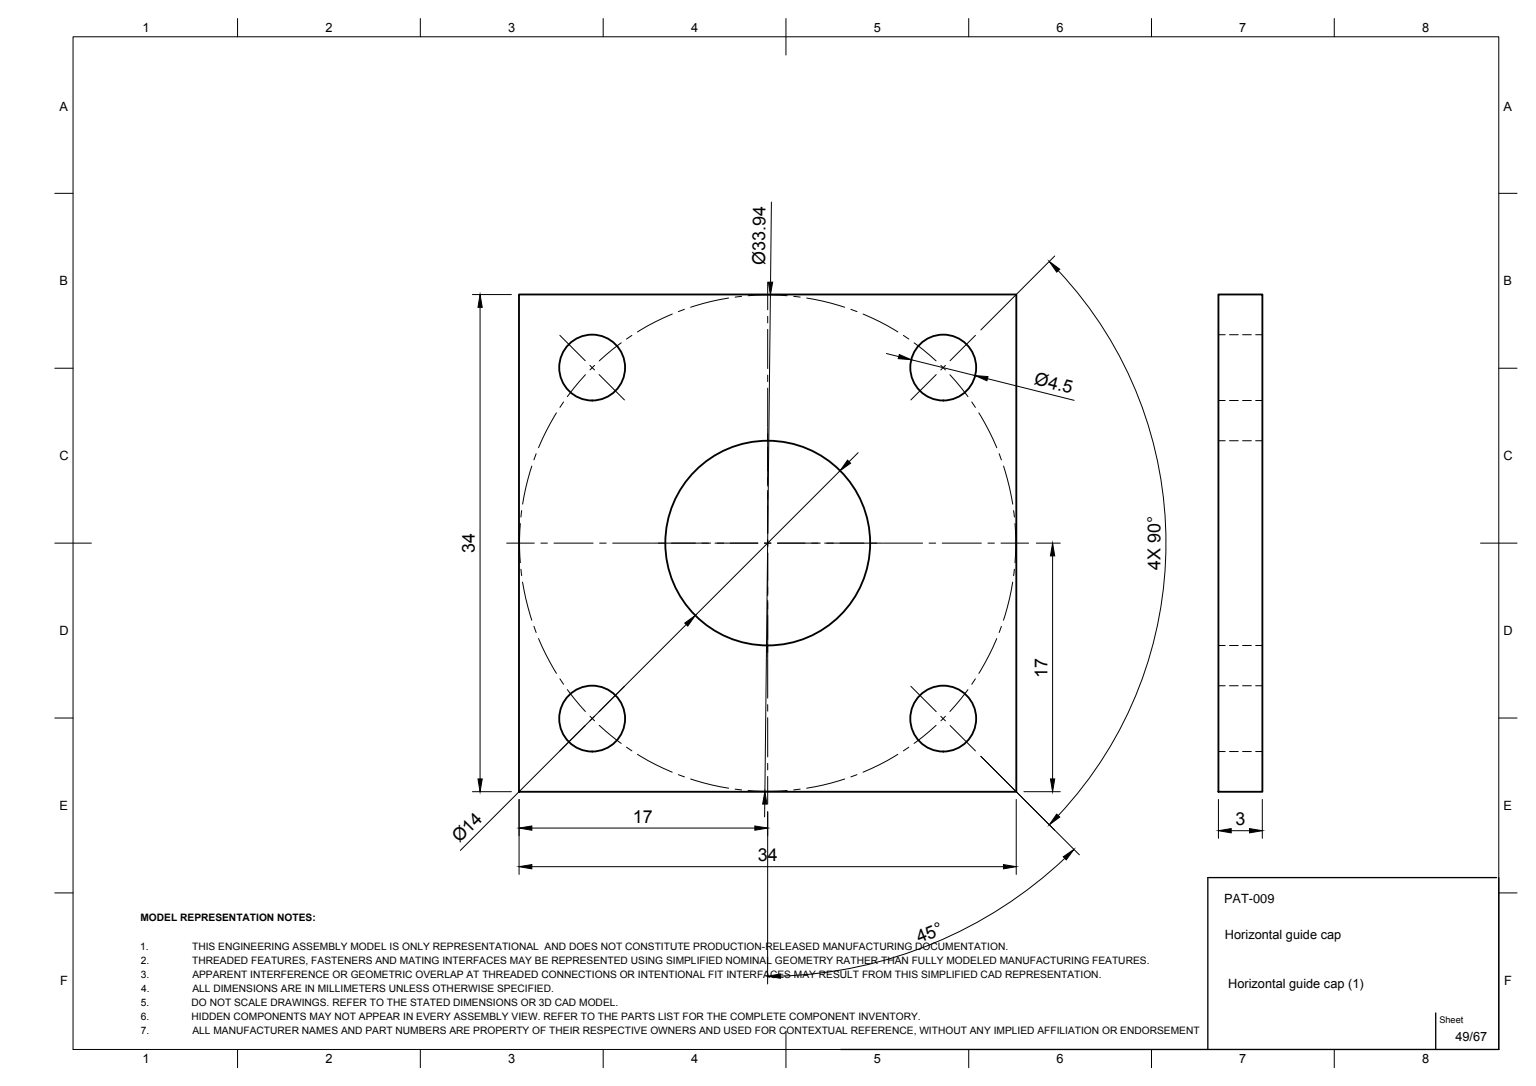
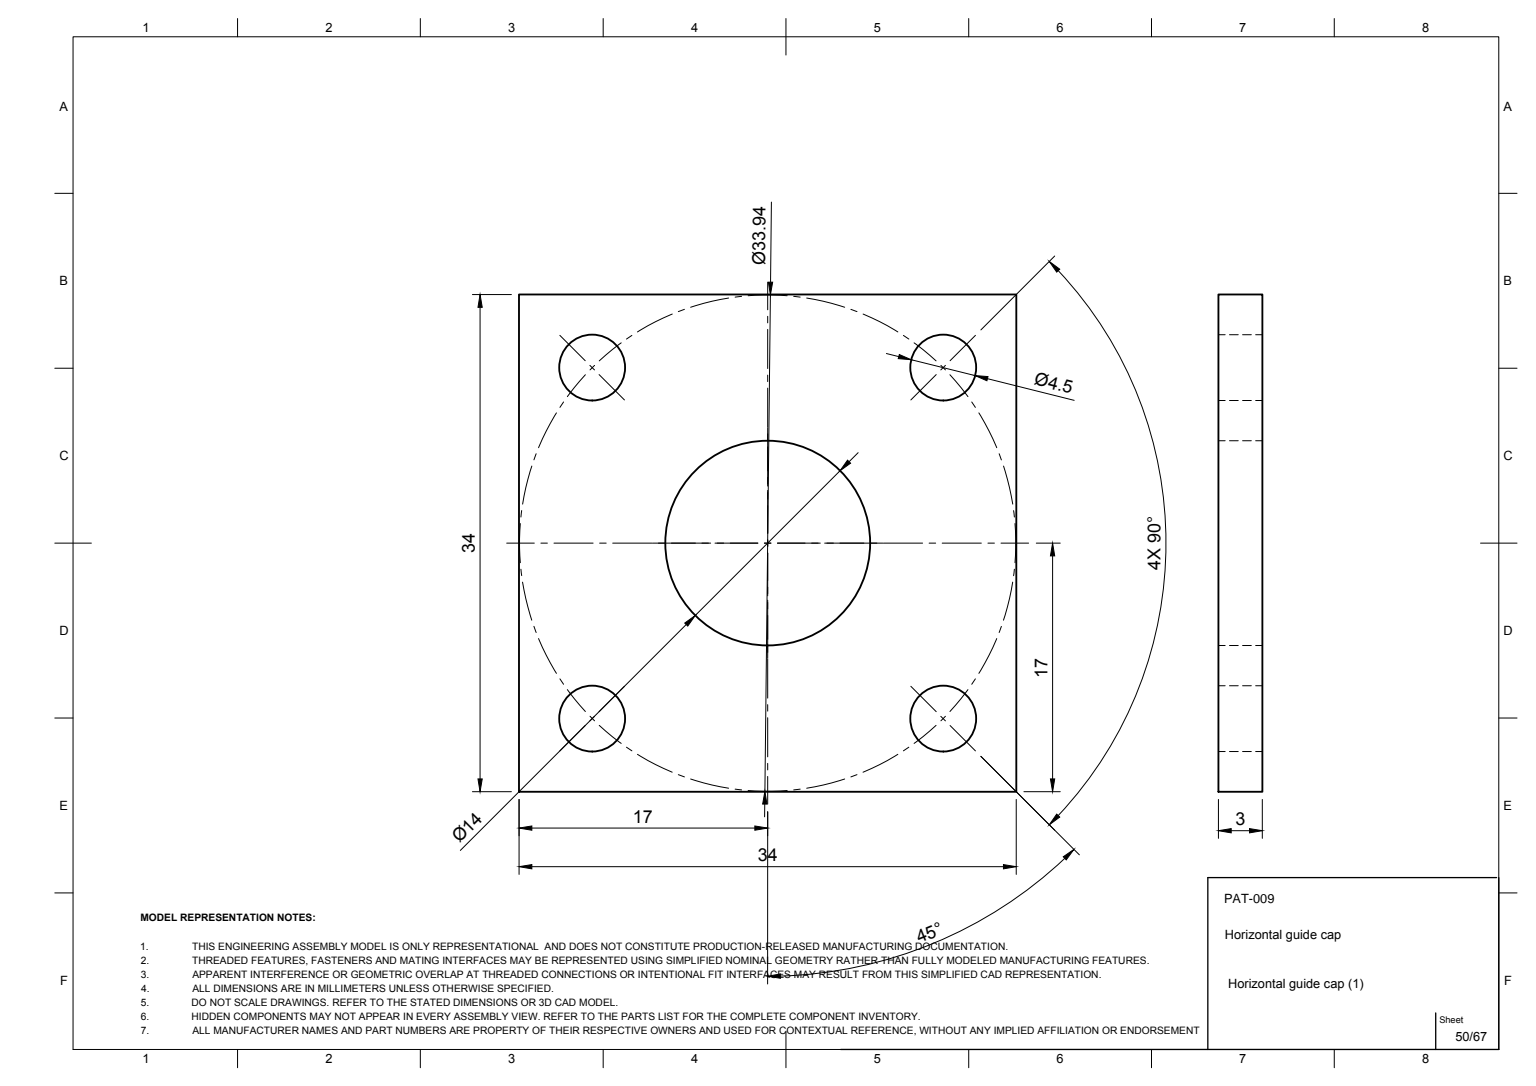
ISO-10303-21;
HEADER;
/* Generated by software containing ST-Developer
 * from STEP Tools, Inc. (www.steptools.com) 
 */

FILE_DESCRIPTION(
/* description */ ('Bell-crank linkage with push rods'),
/* implementation_level */ '2;1');

FILE_NAME(
/* name */ 'Horizontal guide cap.step',
/* time_stamp */ '2026-10-28T03:25:15-07:00',
/* author */ (''),
/* organization */ (''),
/* preprocessor_version */ 'ST-DEVELOPER v20.2',
/* originating_system */ 'Autodesk Translation Framework v15.17.0.0',
/* authorisation */ '');

FILE_SCHEMA (('AUTOMOTIVE_DESIGN { 1 0 10303 214 3 1 1 }'));
ENDSEC;

DATA;
#10=MECHANICAL_DESIGN_GEOMETRIC_PRESENTATION_REPRESENTATION('',(#650),#16678);
#534=SHAPE_REPRESENTATION_RELATIONSHIP('SRR','None',#16955,#588);
#588=ADVANCED_BREP_SHAPE_REPRESENTATION('',(#710),#16660);
#650=STYLED_ITEM('',(#17284),#710);
#710=MANIFOLD_SOLID_BREP('Body1',#8842);
#885=FACE_BOUND('',#2318,.T.);
#886=FACE_BOUND('',#2319,.T.);
#887=FACE_BOUND('',#2320,.T.);
#888=FACE_BOUND('',#2321,.T.);
#889=FACE_BOUND('',#2322,.T.);
#890=FACE_BOUND('',#2325,.T.);
#891=FACE_BOUND('',#2326,.T.);
#892=FACE_BOUND('',#2327,.T.);
#893=FACE_BOUND('',#2328,.T.);
#894=FACE_BOUND('',#2329,.T.);
#1166=PLANE('',#10277);
#1167=PLANE('',#10278);
#1168=PLANE('',#10279);
#1169=PLANE('',#10280);
#1170=PLANE('',#10281);
#1171=PLANE('',#10282);
#1629=FACE_OUTER_BOUND('',#2311,.T.);
#1630=FACE_OUTER_BOUND('',#2312,.T.);
#1631=FACE_OUTER_BOUND('',#2313,.T.);
#1632=FACE_OUTER_BOUND('',#2314,.T.);
#1633=FACE_OUTER_BOUND('',#2315,.T.);
#1634=FACE_OUTER_BOUND('',#2316,.T.);
#1635=FACE_OUTER_BOUND('',#2317,.T.);
#1636=FACE_OUTER_BOUND('',#2323,.T.);
#1637=FACE_OUTER_BOUND('',#2324,.T.);
#1638=FACE_OUTER_BOUND('',#2330,.T.);
#1639=FACE_OUTER_BOUND('',#2331,.T.);
#2311=EDGE_LOOP('',(#7515,#7516,#7517,#7518));
#2312=EDGE_LOOP('',(#7519,#7520,#7521,#7522));
#2313=EDGE_LOOP('',(#7523,#7524,#7525,#7526));
#2314=EDGE_LOOP('',(#7527,#7528,#7529,#7530));
#2315=EDGE_LOOP('',(#7531,#7532,#7533,#7534));
#2316=EDGE_LOOP('',(#7535,#7536,#7537,#7538));
#2317=EDGE_LOOP('',(#7539,#7540,#7541,#7542));
#2318=EDGE_LOOP('',(#7543));
#2319=EDGE_LOOP('',(#7544));
#2320=EDGE_LOOP('',(#7545));
#2321=EDGE_LOOP('',(#7546));
#2322=EDGE_LOOP('',(#7547));
#2323=EDGE_LOOP('',(#7548,#7549,#7550,#7551));
#2324=EDGE_LOOP('',(#7552,#7553,#7554,#7555));
#2325=EDGE_LOOP('',(#7556));
#2326=EDGE_LOOP('',(#7557));
#2327=EDGE_LOOP('',(#7558));
#2328=EDGE_LOOP('',(#7559));
#2329=EDGE_LOOP('',(#7560));
#2330=EDGE_LOOP('',(#7561,#7562,#7563,#7564));
#2331=EDGE_LOOP('',(#7565,#7566,#7567,#7568));
#2926=LINE('',#15849,#3475);
#2927=LINE('',#15855,#3476);
#2928=LINE('',#15861,#3477);
#2929=LINE('',#15867,#3478);
#2930=LINE('',#15873,#3479);
#2931=LINE('',#15878,#3480);
#2932=LINE('',#15880,#3481);
#2933=LINE('',#15882,#3482);
#2934=LINE('',#15883,#3483);
#2935=LINE('',#15886,#3484);
#2936=LINE('',#15888,#3485);
#2937=LINE('',#15889,#3486);
#2938=LINE('',#15892,#3487);
#2939=LINE('',#15894,#3488);
#2940=LINE('',#15895,#3489);
#2941=LINE('',#15897,#3490);
#2942=LINE('',#15898,#3491);
#3475=VECTOR('',#12644,0.225);
#3476=VECTOR('',#12651,0.225);
#3477=VECTOR('',#12658,0.225);
#3478=VECTOR('',#12665,0.225);
#3479=VECTOR('',#12672,0.7);
#3480=VECTOR('',#12677,1.);
#3481=VECTOR('',#12678,1.);
#3482=VECTOR('',#12679,1.);
#3483=VECTOR('',#12680,1.);
#3484=VECTOR('',#12683,1.);
#3485=VECTOR('',#12684,1.);
#3486=VECTOR('',#12685,1.);
#3487=VECTOR('',#12688,1.);
#3488=VECTOR('',#12689,1.);
#3489=VECTOR('',#12690,1.);
#3490=VECTOR('',#12693,1.);
#3491=VECTOR('',#12694,1.);
#3999=CIRCLE('',#10263,0.225);
#4000=CIRCLE('',#10264,0.225);
#4001=CIRCLE('',#10266,0.225);
#4002=CIRCLE('',#10267,0.225);
#4003=CIRCLE('',#10269,0.225);
#4004=CIRCLE('',#10270,0.225);
#4005=CIRCLE('',#10272,0.225);
#4006=CIRCLE('',#10273,0.225);
#4007=CIRCLE('',#10275,0.7);
#4008=CIRCLE('',#10276,0.7);
#4650=VERTEX_POINT('',#15846);
#4651=VERTEX_POINT('',#15848);
#4652=VERTEX_POINT('',#15852);
#4653=VERTEX_POINT('',#15854);
#4654=VERTEX_POINT('',#15858);
#4655=VERTEX_POINT('',#15860);
#4656=VERTEX_POINT('',#15864);
#4657=VERTEX_POINT('',#15866);
#4658=VERTEX_POINT('',#15870);
#4659=VERTEX_POINT('',#15872);
#4660=VERTEX_POINT('',#15876);
#4661=VERTEX_POINT('',#15877);
#4662=VERTEX_POINT('',#15879);
#4663=VERTEX_POINT('',#15881);
#4664=VERTEX_POINT('',#15885);
#4665=VERTEX_POINT('',#15887);
#4666=VERTEX_POINT('',#15891);
#4667=VERTEX_POINT('',#15893);
#5635=EDGE_CURVE('',#4650,#4650,#3999,.T.);
#5636=EDGE_CURVE('',#4650,#4651,#2926,.T.);
#5637=EDGE_CURVE('',#4651,#4651,#4000,.T.);
#5638=EDGE_CURVE('',#4652,#4652,#4001,.T.);
#5639=EDGE_CURVE('',#4652,#4653,#2927,.T.);
#5640=EDGE_CURVE('',#4653,#4653,#4002,.T.);
#5641=EDGE_CURVE('',#4654,#4654,#4003,.T.);
#5642=EDGE_CURVE('',#4654,#4655,#2928,.T.);
#5643=EDGE_CURVE('',#4655,#4655,#4004,.T.);
#5644=EDGE_CURVE('',#4656,#4656,#4005,.T.);
#5645=EDGE_CURVE('',#4656,#4657,#2929,.T.);
#5646=EDGE_CURVE('',#4657,#4657,#4006,.T.);
#5647=EDGE_CURVE('',#4658,#4658,#4007,.T.);
#5648=EDGE_CURVE('',#4658,#4659,#2930,.T.);
#5649=EDGE_CURVE('',#4659,#4659,#4008,.T.);
#5650=EDGE_CURVE('',#4660,#4661,#2931,.T.);
#5651=EDGE_CURVE('',#4661,#4662,#2932,.T.);
#5652=EDGE_CURVE('',#4663,#4662,#2933,.T.);
#5653=EDGE_CURVE('',#4660,#4663,#2934,.T.);
#5654=EDGE_CURVE('',#4664,#4660,#2935,.T.);
#5655=EDGE_CURVE('',#4665,#4663,#2936,.T.);
#5656=EDGE_CURVE('',#4664,#4665,#2937,.T.);
#5657=EDGE_CURVE('',#4666,#4664,#2938,.T.);
#5658=EDGE_CURVE('',#4667,#4665,#2939,.T.);
#5659=EDGE_CURVE('',#4666,#4667,#2940,.T.);
#5660=EDGE_CURVE('',#4661,#4666,#2941,.T.);
#5661=EDGE_CURVE('',#4662,#4667,#2942,.T.);
#7515=ORIENTED_EDGE('',*,*,#5635,.F.);
#7516=ORIENTED_EDGE('',*,*,#5636,.T.);
#7517=ORIENTED_EDGE('',*,*,#5637,.F.);
#7518=ORIENTED_EDGE('',*,*,#5636,.F.);
#7519=ORIENTED_EDGE('',*,*,#5638,.F.);
#7520=ORIENTED_EDGE('',*,*,#5639,.T.);
#7521=ORIENTED_EDGE('',*,*,#5640,.F.);
#7522=ORIENTED_EDGE('',*,*,#5639,.F.);
#7523=ORIENTED_EDGE('',*,*,#5641,.F.);
#7524=ORIENTED_EDGE('',*,*,#5642,.T.);
#7525=ORIENTED_EDGE('',*,*,#5643,.F.);
#7526=ORIENTED_EDGE('',*,*,#5642,.F.);
#7527=ORIENTED_EDGE('',*,*,#5644,.F.);
#7528=ORIENTED_EDGE('',*,*,#5645,.T.);
#7529=ORIENTED_EDGE('',*,*,#5646,.F.);
#7530=ORIENTED_EDGE('',*,*,#5645,.F.);
#7531=ORIENTED_EDGE('',*,*,#5647,.F.);
#7532=ORIENTED_EDGE('',*,*,#5648,.T.);
#7533=ORIENTED_EDGE('',*,*,#5649,.F.);
#7534=ORIENTED_EDGE('',*,*,#5648,.F.);
#7535=ORIENTED_EDGE('',*,*,#5650,.T.);
#7536=ORIENTED_EDGE('',*,*,#5651,.T.);
#7537=ORIENTED_EDGE('',*,*,#5652,.F.);
#7538=ORIENTED_EDGE('',*,*,#5653,.F.);
#7539=ORIENTED_EDGE('',*,*,#5654,.T.);
#7540=ORIENTED_EDGE('',*,*,#5653,.T.);
#7541=ORIENTED_EDGE('',*,*,#5655,.F.);
#7542=ORIENTED_EDGE('',*,*,#5656,.F.);
#7543=ORIENTED_EDGE('',*,*,#5649,.T.);
#7544=ORIENTED_EDGE('',*,*,#5646,.T.);
#7545=ORIENTED_EDGE('',*,*,#5643,.T.);
#7546=ORIENTED_EDGE('',*,*,#5640,.T.);
#7547=ORIENTED_EDGE('',*,*,#5637,.T.);
#7548=ORIENTED_EDGE('',*,*,#5657,.T.);
#7549=ORIENTED_EDGE('',*,*,#5656,.T.);
#7550=ORIENTED_EDGE('',*,*,#5658,.F.);
#7551=ORIENTED_EDGE('',*,*,#5659,.F.);
#7552=ORIENTED_EDGE('',*,*,#5660,.T.);
#7553=ORIENTED_EDGE('',*,*,#5659,.T.);
#7554=ORIENTED_EDGE('',*,*,#5661,.F.);
#7555=ORIENTED_EDGE('',*,*,#5651,.F.);
#7556=ORIENTED_EDGE('',*,*,#5647,.T.);
#7557=ORIENTED_EDGE('',*,*,#5644,.T.);
#7558=ORIENTED_EDGE('',*,*,#5641,.T.);
#7559=ORIENTED_EDGE('',*,*,#5638,.T.);
#7560=ORIENTED_EDGE('',*,*,#5635,.T.);
#7561=ORIENTED_EDGE('',*,*,#5661,.T.);
#7562=ORIENTED_EDGE('',*,*,#5658,.T.);
#7563=ORIENTED_EDGE('',*,*,#5655,.T.);
#7564=ORIENTED_EDGE('',*,*,#5652,.T.);
#7565=ORIENTED_EDGE('',*,*,#5660,.F.);
#7566=ORIENTED_EDGE('',*,*,#5650,.F.);
#7567=ORIENTED_EDGE('',*,*,#5654,.F.);
#7568=ORIENTED_EDGE('',*,*,#5657,.F.);
#8216=CYLINDRICAL_SURFACE('',#10262,0.225);
#8217=CYLINDRICAL_SURFACE('',#10265,0.225);
#8218=CYLINDRICAL_SURFACE('',#10268,0.225);
#8219=CYLINDRICAL_SURFACE('',#10271,0.225);
#8220=CYLINDRICAL_SURFACE('',#10274,0.7);
#8654=ADVANCED_FACE('',(#1629),#8216,.F.);
#8655=ADVANCED_FACE('',(#1630),#8217,.F.);
#8656=ADVANCED_FACE('',(#1631),#8218,.F.);
#8657=ADVANCED_FACE('',(#1632),#8219,.F.);
#8658=ADVANCED_FACE('',(#1633),#8220,.F.);
#8659=ADVANCED_FACE('',(#1634),#1166,.T.);
#8660=ADVANCED_FACE('',(#1635,#885,#886,#887,#888,#889),#1167,.T.);
#8661=ADVANCED_FACE('',(#1636),#1168,.T.);
#8662=ADVANCED_FACE('',(#1637,#890,#891,#892,#893,#894),#1169,.T.);
#8663=ADVANCED_FACE('',(#1638),#1170,.T.);
#8664=ADVANCED_FACE('',(#1639),#1171,.F.);
#8842=CLOSED_SHELL('',(#8654,#8655,#8656,#8657,#8658,#8659,#8660,#8661,
#8662,#8663,#8664));
#10261=AXIS2_PLACEMENT_3D('',#15844,#12638,#12639);
#10262=AXIS2_PLACEMENT_3D('',#15845,#12640,#12641);
#10263=AXIS2_PLACEMENT_3D('',#15847,#12642,#12643);
#10264=AXIS2_PLACEMENT_3D('',#15850,#12645,#12646);
#10265=AXIS2_PLACEMENT_3D('',#15851,#12647,#12648);
#10266=AXIS2_PLACEMENT_3D('',#15853,#12649,#12650);
#10267=AXIS2_PLACEMENT_3D('',#15856,#12652,#12653);
#10268=AXIS2_PLACEMENT_3D('',#15857,#12654,#12655);
#10269=AXIS2_PLACEMENT_3D('',#15859,#12656,#12657);
#10270=AXIS2_PLACEMENT_3D('',#15862,#12659,#12660);
#10271=AXIS2_PLACEMENT_3D('',#15863,#12661,#12662);
#10272=AXIS2_PLACEMENT_3D('',#15865,#12663,#12664);
#10273=AXIS2_PLACEMENT_3D('',#15868,#12666,#12667);
#10274=AXIS2_PLACEMENT_3D('',#15869,#12668,#12669);
#10275=AXIS2_PLACEMENT_3D('',#15871,#12670,#12671);
#10276=AXIS2_PLACEMENT_3D('',#15874,#12673,#12674);
#10277=AXIS2_PLACEMENT_3D('',#15875,#12675,#12676);
#10278=AXIS2_PLACEMENT_3D('',#15884,#12681,#12682);
#10279=AXIS2_PLACEMENT_3D('',#15890,#12686,#12687);
#10280=AXIS2_PLACEMENT_3D('',#15896,#12691,#12692);
#10281=AXIS2_PLACEMENT_3D('',#15899,#12695,#12696);
#10282=AXIS2_PLACEMENT_3D('',#15900,#12697,#12698);
#12638=DIRECTION('axis',(0.,0.,1.));
#12639=DIRECTION('refdir',(1.,0.,0.));
#12640=DIRECTION('center_axis',(1.,0.,0.));
#12641=DIRECTION('ref_axis',(0.,0.,-1.));
#12642=DIRECTION('center_axis',(1.,0.,0.));
#12643=DIRECTION('ref_axis',(0.,0.,-1.));
#12644=DIRECTION('',(1.,0.,0.));
#12645=DIRECTION('center_axis',(-1.,0.,0.));
#12646=DIRECTION('ref_axis',(0.,0.,-1.));
#12647=DIRECTION('center_axis',(1.,0.,0.));
#12648=DIRECTION('ref_axis',(0.,0.,-1.));
#12649=DIRECTION('center_axis',(1.,0.,0.));
#12650=DIRECTION('ref_axis',(0.,0.,-1.));
#12651=DIRECTION('',(1.,0.,0.));
#12652=DIRECTION('center_axis',(-1.,0.,0.));
#12653=DIRECTION('ref_axis',(0.,0.,-1.));
#12654=DIRECTION('center_axis',(1.,0.,0.));
#12655=DIRECTION('ref_axis',(0.,0.,-1.));
#12656=DIRECTION('center_axis',(1.,0.,0.));
#12657=DIRECTION('ref_axis',(0.,0.,-1.));
#12658=DIRECTION('',(1.,0.,0.));
#12659=DIRECTION('center_axis',(-1.,0.,0.));
#12660=DIRECTION('ref_axis',(0.,0.,-1.));
#12661=DIRECTION('center_axis',(1.,0.,0.));
#12662=DIRECTION('ref_axis',(0.,0.,-1.));
#12663=DIRECTION('center_axis',(1.,0.,0.));
#12664=DIRECTION('ref_axis',(0.,0.,-1.));
#12665=DIRECTION('',(1.,0.,0.));
#12666=DIRECTION('center_axis',(-1.,0.,0.));
#12667=DIRECTION('ref_axis',(0.,0.,-1.));
#12668=DIRECTION('center_axis',(1.,0.,0.));
#12669=DIRECTION('ref_axis',(0.,0.,-1.));
#12670=DIRECTION('center_axis',(1.,0.,0.));
#12671=DIRECTION('ref_axis',(0.,0.,-1.));
#12672=DIRECTION('',(1.,0.,0.));
#12673=DIRECTION('center_axis',(-1.,0.,0.));
#12674=DIRECTION('ref_axis',(0.,0.,-1.));
#12675=DIRECTION('center_axis',(0.,1.,0.));
#12676=DIRECTION('ref_axis',(-1.,0.,0.));
#12677=DIRECTION('',(-1.,0.,0.));
#12678=DIRECTION('',(0.,0.,1.));
#12679=DIRECTION('',(-1.,0.,0.));
#12680=DIRECTION('',(0.,0.,1.));
#12681=DIRECTION('center_axis',(1.,0.,0.));
#12682=DIRECTION('ref_axis',(0.,1.,0.));
#12683=DIRECTION('',(0.,1.,0.));
#12684=DIRECTION('',(0.,1.,0.));
#12685=DIRECTION('',(0.,0.,1.));
#12686=DIRECTION('center_axis',(0.,-1.,0.));
#12687=DIRECTION('ref_axis',(1.,0.,0.));
#12688=DIRECTION('',(1.,0.,0.));
#12689=DIRECTION('',(1.,0.,0.));
#12690=DIRECTION('',(0.,0.,1.));
#12691=DIRECTION('center_axis',(-1.,0.,0.));
#12692=DIRECTION('ref_axis',(0.,-1.,0.));
#12693=DIRECTION('',(0.,-1.,0.));
#12694=DIRECTION('',(0.,-1.,0.));
#12695=DIRECTION('center_axis',(0.,0.,1.));
#12696=DIRECTION('ref_axis',(1.,0.,0.));
#12697=DIRECTION('center_axis',(0.,0.,1.));
#12698=DIRECTION('ref_axis',(1.,0.,0.));
#15844=CARTESIAN_POINT('',(0.,0.,0.));
#15845=CARTESIAN_POINT('Origin',(8.1,3.2,2.8));
#15846=CARTESIAN_POINT('',(8.2,3.2,3.025));
#15847=CARTESIAN_POINT('Origin',(8.2,3.2,2.8));
#15848=CARTESIAN_POINT('',(8.5,3.2,3.025));
#15849=CARTESIAN_POINT('',(8.1,3.2,3.025));
#15850=CARTESIAN_POINT('Origin',(8.5,3.2,2.8));
#15851=CARTESIAN_POINT('Origin',(8.1,0.8,5.2));
#15852=CARTESIAN_POINT('',(8.2,0.8,5.425));
#15853=CARTESIAN_POINT('Origin',(8.2,0.8,5.2));
#15854=CARTESIAN_POINT('',(8.5,0.8,5.425));
#15855=CARTESIAN_POINT('',(8.1,0.8,5.425));
#15856=CARTESIAN_POINT('Origin',(8.5,0.8,5.2));
#15857=CARTESIAN_POINT('Origin',(8.1,0.8,2.8));
#15858=CARTESIAN_POINT('',(8.2,0.8,3.025));
#15859=CARTESIAN_POINT('Origin',(8.2,0.8,2.8));
#15860=CARTESIAN_POINT('',(8.5,0.8,3.025));
#15861=CARTESIAN_POINT('',(8.1,0.8,3.025));
#15862=CARTESIAN_POINT('Origin',(8.5,0.8,2.8));
#15863=CARTESIAN_POINT('Origin',(8.1,3.2,5.2));
#15864=CARTESIAN_POINT('',(8.2,3.2,5.425));
#15865=CARTESIAN_POINT('Origin',(8.2,3.2,5.2));
#15866=CARTESIAN_POINT('',(8.5,3.2,5.425));
#15867=CARTESIAN_POINT('',(8.1,3.2,5.425));
#15868=CARTESIAN_POINT('Origin',(8.5,3.2,5.2));
#15869=CARTESIAN_POINT('Origin',(8.1,2.,4.));
#15870=CARTESIAN_POINT('',(8.2,2.,4.7));
#15871=CARTESIAN_POINT('Origin',(8.2,2.,4.));
#15872=CARTESIAN_POINT('',(8.5,2.,4.7));
#15873=CARTESIAN_POINT('',(8.1,2.,4.7));
#15874=CARTESIAN_POINT('Origin',(8.5,2.,4.));
#15875=CARTESIAN_POINT('Origin',(8.5,3.7,2.3));
#15876=CARTESIAN_POINT('',(8.5,3.7,2.3));
#15877=CARTESIAN_POINT('',(8.2,3.7,2.3));
#15878=CARTESIAN_POINT('',(8.5,3.7,2.3));
#15879=CARTESIAN_POINT('',(8.2,3.7,5.7));
#15880=CARTESIAN_POINT('',(8.2,3.7,2.3));
#15881=CARTESIAN_POINT('',(8.5,3.7,5.7));
#15882=CARTESIAN_POINT('',(8.5,3.7,5.7));
#15883=CARTESIAN_POINT('',(8.5,3.7,2.3));
#15884=CARTESIAN_POINT('Origin',(8.5,0.3,2.3));
#15885=CARTESIAN_POINT('',(8.5,0.3,2.3));
#15886=CARTESIAN_POINT('',(8.5,0.3,2.3));
#15887=CARTESIAN_POINT('',(8.5,0.3,5.7));
#15888=CARTESIAN_POINT('',(8.5,0.3,5.7));
#15889=CARTESIAN_POINT('',(8.5,0.3,2.3));
#15890=CARTESIAN_POINT('Origin',(8.2,0.3,2.3));
#15891=CARTESIAN_POINT('',(8.2,0.3,2.3));
#15892=CARTESIAN_POINT('',(8.2,0.3,2.3));
#15893=CARTESIAN_POINT('',(8.2,0.3,5.7));
#15894=CARTESIAN_POINT('',(8.2,0.3,5.7));
#15895=CARTESIAN_POINT('',(8.2,0.3,2.3));
#15896=CARTESIAN_POINT('Origin',(8.2,3.7,2.3));
#15897=CARTESIAN_POINT('',(8.2,3.7,2.3));
#15898=CARTESIAN_POINT('',(8.2,3.7,5.7));
#15899=CARTESIAN_POINT('Origin',(8.35,2.,5.7));
#15900=CARTESIAN_POINT('Origin',(8.35,2.,2.3));
#16596=UNCERTAINTY_MEASURE_WITH_UNIT(LENGTH_MEASURE(0.001),#16679,
'DISTANCE_ACCURACY_VALUE',
'Maximum model space distance between geometric entities at asserted c
onnectivities');
#16614=UNCERTAINTY_MEASURE_WITH_UNIT(LENGTH_MEASURE(0.001),#16679,
'DISTANCE_ACCURACY_VALUE',
'Maximum model space distance between geometric entities at asserted c
onnectivities');
#16660=(
GEOMETRIC_REPRESENTATION_CONTEXT(3)
GLOBAL_UNCERTAINTY_ASSIGNED_CONTEXT((#16596))
GLOBAL_UNIT_ASSIGNED_CONTEXT((#16679,#16681,#16682))
REPRESENTATION_CONTEXT('','3D')
);
#16678=(
GEOMETRIC_REPRESENTATION_CONTEXT(3)
GLOBAL_UNCERTAINTY_ASSIGNED_CONTEXT((#16614))
GLOBAL_UNIT_ASSIGNED_CONTEXT((#16679,#16681,#16682))
REPRESENTATION_CONTEXT('','3D')
);
#16679=(
LENGTH_UNIT()
NAMED_UNIT(*)
SI_UNIT(.CENTI.,.METRE.)
);
#16681=(
NAMED_UNIT(*)
PLANE_ANGLE_UNIT()
SI_UNIT($,.RADIAN.)
);
#16682=(
NAMED_UNIT(*)
SI_UNIT($,.STERADIAN.)
SOLID_ANGLE_UNIT()
);
#16728=SHAPE_DEFINITION_REPRESENTATION(#16802,#16955);
#16802=PRODUCT_DEFINITION_SHAPE('',$,#17019);
#16955=SHAPE_REPRESENTATION('',(#10261),#16660);
#16973=PRODUCT_DEFINITION_CONTEXT('part definition',#17164,'design');
#17019=PRODUCT_DEFINITION('Horizontal guide cap','Horizontal guide cap',
#17082,#16973);
#17082=PRODUCT_DEFINITION_FORMATION('',$,#17211);
#17164=APPLICATION_CONTEXT(
'Core Data for Automotive Mechanical Design Process');
#17165=PRODUCT_CONTEXT('part definition',#17164,'mechanical');
#17211=PRODUCT('Horizontal guide cap','Horizontal guide cap',
'Horizontal guide cap',(#17165));
#17278=COLOUR_RGB('Sky Blue',0.24,0.69,0.87);
#17279=FILL_AREA_STYLE_COLOUR('',#17278);
#17280=FILL_AREA_STYLE('',(#17279));
#17281=SURFACE_STYLE_FILL_AREA(#17280);
#17282=SURFACE_SIDE_STYLE('',(#17281));
#17283=SURFACE_STYLE_USAGE(.BOTH.,#17282);
#17284=PRESENTATION_STYLE_ASSIGNMENT((#17283));
ENDSEC;
END-ISO-10303-21;
